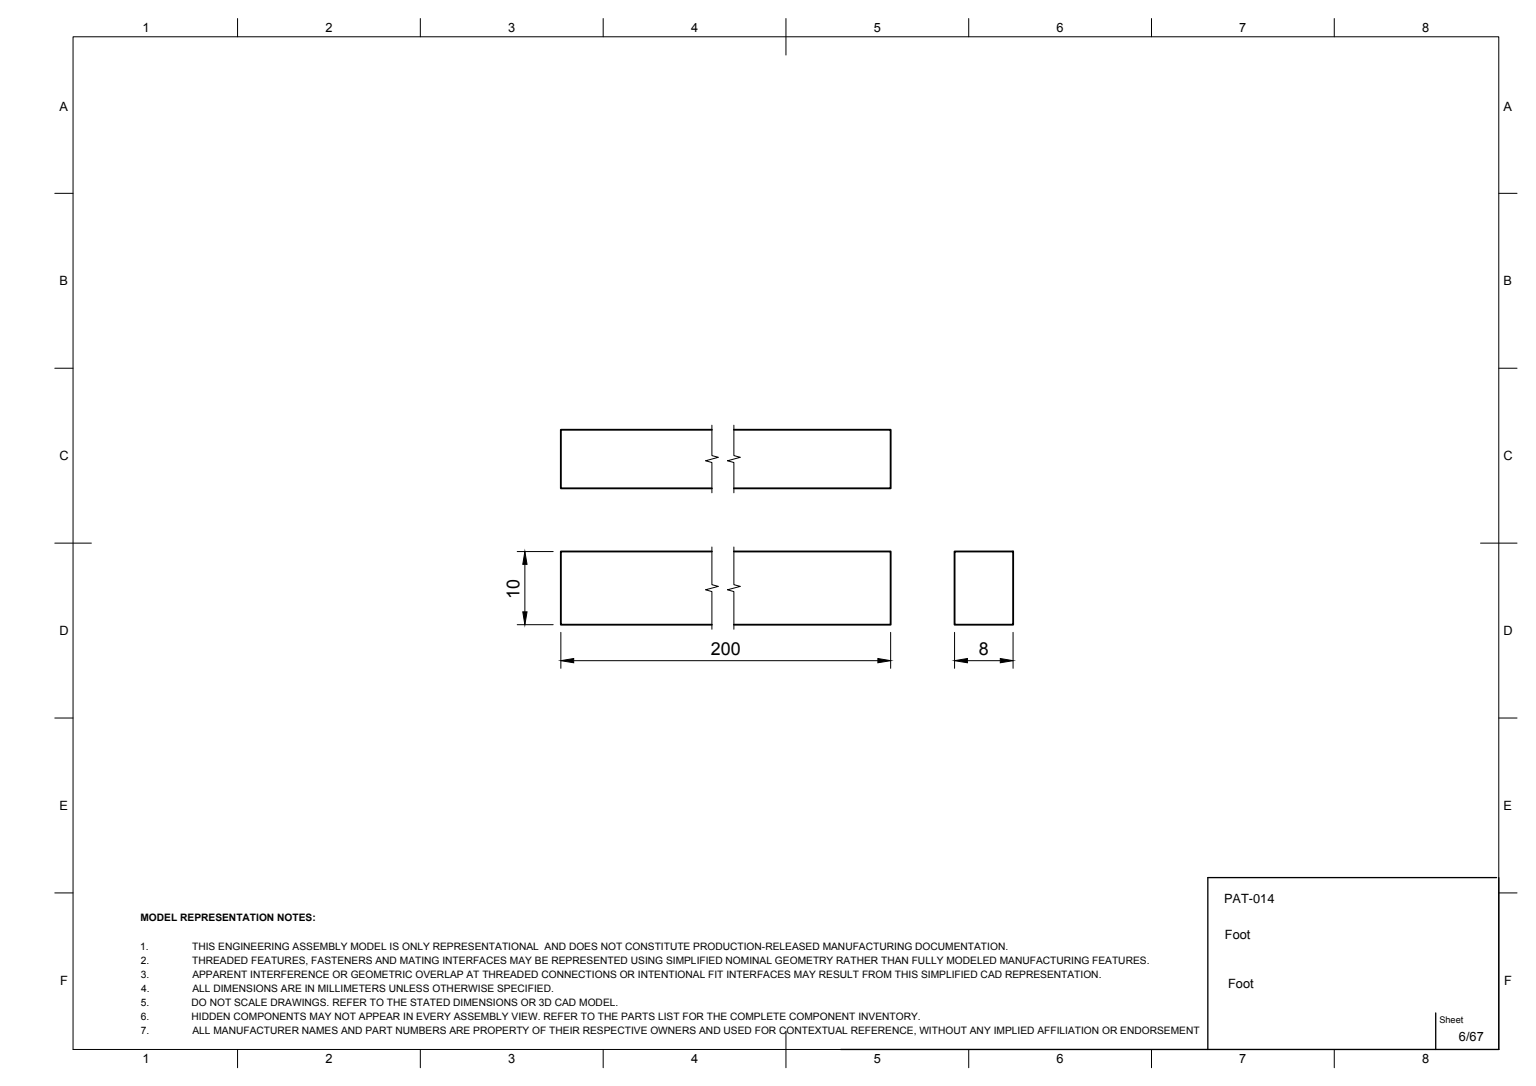
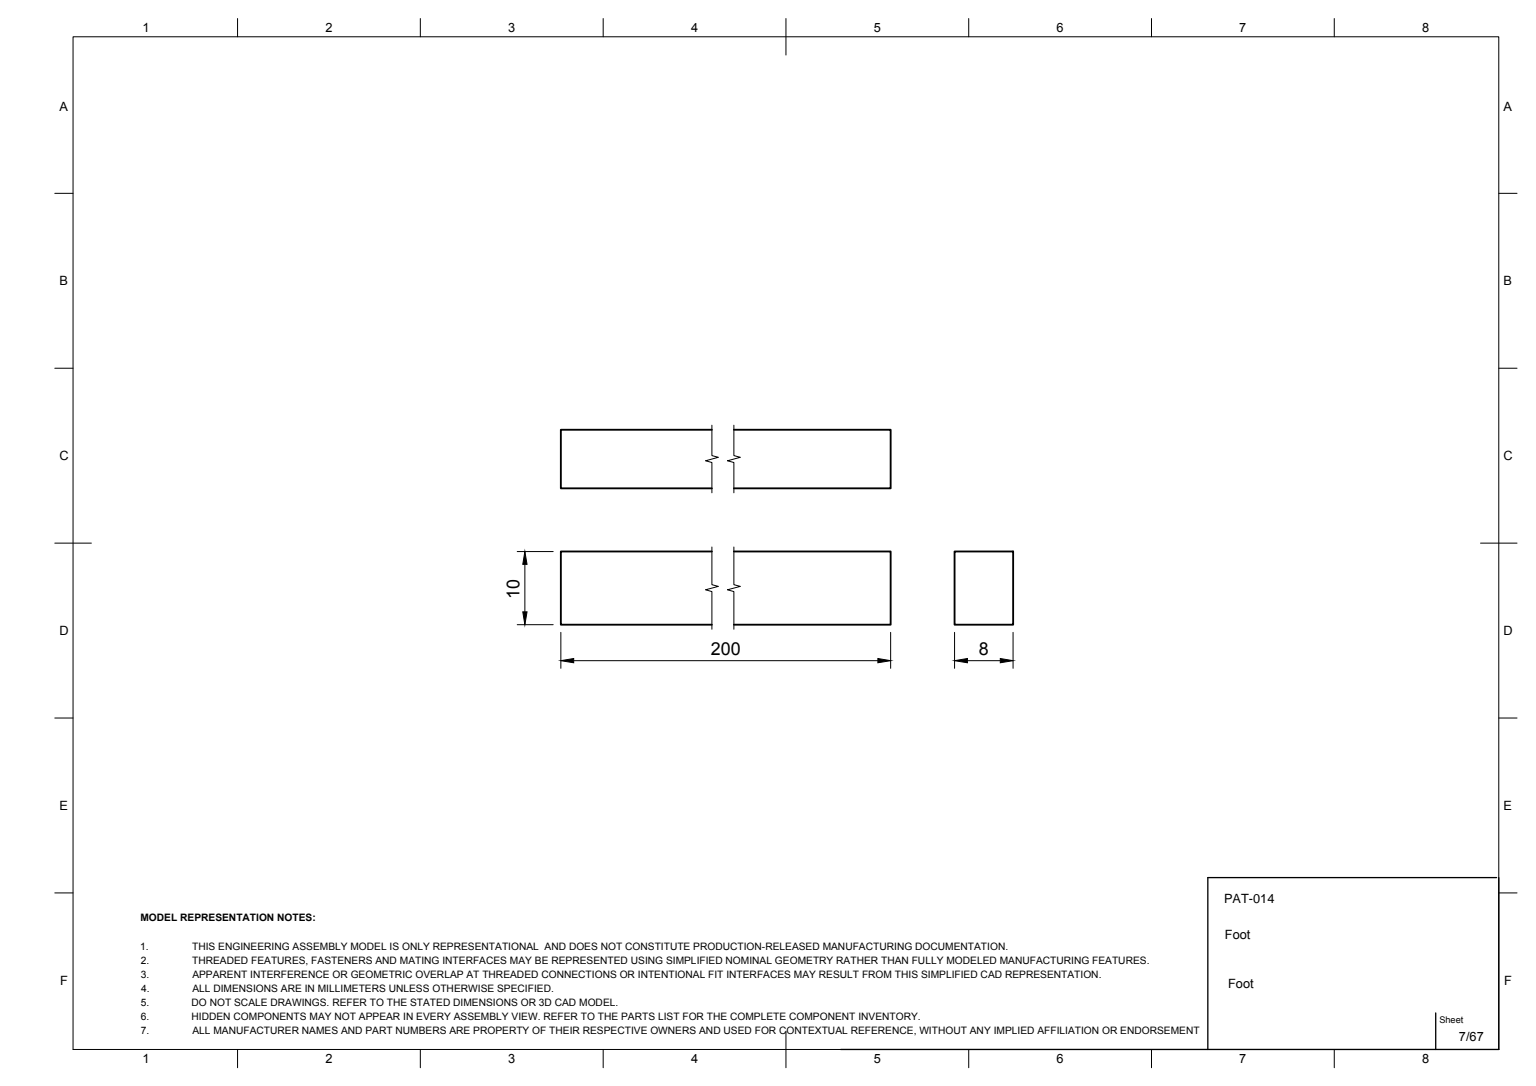
ISO-10303-21;
HEADER;
/* Generated by software containing ST-Developer
 * from STEP Tools, Inc. (www.steptools.com) 
 */

FILE_DESCRIPTION(
/* description */ ('Bin tilter linkage'),
/* implementation_level */ '2;1');

FILE_NAME(
/* name */ 'Foot.step',
/* time_stamp */ '2026-10-28T03:26:24-07:00',
/* author */ (''),
/* organization */ (''),
/* preprocessor_version */ 'ST-DEVELOPER v20.2',
/* originating_system */ 'Autodesk Translation Framework v15.17.0.0',
/* authorisation */ '');

FILE_SCHEMA (('AUTOMOTIVE_DESIGN { 1 0 10303 214 3 1 1 }'));
ENDSEC;

DATA;
#10=MECHANICAL_DESIGN_GEOMETRIC_PRESENTATION_REPRESENTATION('',(#863),#23728);
#651=SHAPE_REPRESENTATION_RELATIONSHIP('SRR','None',#24115,#757);
#757=ADVANCED_BREP_SHAPE_REPRESENTATION('',(#977),#23615);
#863=STYLED_ITEM('',(#24779),#977);
#977=MANIFOLD_SOLID_BREP('Body1',#12393);
#1498=PLANE('',#13722);
#1499=PLANE('',#13723);
#1500=PLANE('',#13724);
#1501=PLANE('',#13725);
#1502=PLANE('',#13726);
#1503=PLANE('',#13727);
#1908=FACE_OUTER_BOUND('',#2709,.T.);
#1909=FACE_OUTER_BOUND('',#2710,.T.);
#1910=FACE_OUTER_BOUND('',#2711,.T.);
#1911=FACE_OUTER_BOUND('',#2712,.T.);
#1912=FACE_OUTER_BOUND('',#2713,.T.);
#1913=FACE_OUTER_BOUND('',#2714,.T.);
#2709=EDGE_LOOP('',(#8469,#8470,#8471,#8472));
#2710=EDGE_LOOP('',(#8473,#8474,#8475,#8476));
#2711=EDGE_LOOP('',(#8477,#8478,#8479,#8480));
#2712=EDGE_LOOP('',(#8481,#8482,#8483,#8484));
#2713=EDGE_LOOP('',(#8485,#8486,#8487,#8488));
#2714=EDGE_LOOP('',(#8489,#8490,#8491,#8492));
#3873=LINE('',#19850,#4548);
#3874=LINE('',#19852,#4549);
#3875=LINE('',#19854,#4550);
#3876=LINE('',#19855,#4551);
#3877=LINE('',#19858,#4552);
#3878=LINE('',#19860,#4553);
#3879=LINE('',#19861,#4554);
#3880=LINE('',#19864,#4555);
#3881=LINE('',#19866,#4556);
#3882=LINE('',#19867,#4557);
#3883=LINE('',#19869,#4558);
#3884=LINE('',#19870,#4559);
#4548=VECTOR('',#15592,1.);
#4549=VECTOR('',#15593,1.);
#4550=VECTOR('',#15594,1.);
#4551=VECTOR('',#15595,1.);
#4552=VECTOR('',#15598,1.);
#4553=VECTOR('',#15599,1.);
#4554=VECTOR('',#15600,1.);
#4555=VECTOR('',#15603,1.);
#4556=VECTOR('',#15604,1.);
#4557=VECTOR('',#15605,1.);
#4558=VECTOR('',#15608,1.);
#4559=VECTOR('',#15609,1.);
#5989=VERTEX_POINT('',#19848);
#5990=VERTEX_POINT('',#19849);
#5991=VERTEX_POINT('',#19851);
#5992=VERTEX_POINT('',#19853);
#5993=VERTEX_POINT('',#19857);
#5994=VERTEX_POINT('',#19859);
#5995=VERTEX_POINT('',#19863);
#5996=VERTEX_POINT('',#19865);
#6974=EDGE_CURVE('',#5989,#5990,#3873,.T.);
#6975=EDGE_CURVE('',#5990,#5991,#3874,.T.);
#6976=EDGE_CURVE('',#5992,#5991,#3875,.T.);
#6977=EDGE_CURVE('',#5989,#5992,#3876,.T.);
#6978=EDGE_CURVE('',#5993,#5989,#3877,.T.);
#6979=EDGE_CURVE('',#5994,#5992,#3878,.T.);
#6980=EDGE_CURVE('',#5993,#5994,#3879,.T.);
#6981=EDGE_CURVE('',#5995,#5993,#3880,.T.);
#6982=EDGE_CURVE('',#5996,#5994,#3881,.T.);
#6983=EDGE_CURVE('',#5995,#5996,#3882,.T.);
#6984=EDGE_CURVE('',#5990,#5995,#3883,.T.);
#6985=EDGE_CURVE('',#5991,#5996,#3884,.T.);
#8469=ORIENTED_EDGE('',*,*,#6974,.T.);
#8470=ORIENTED_EDGE('',*,*,#6975,.T.);
#8471=ORIENTED_EDGE('',*,*,#6976,.F.);
#8472=ORIENTED_EDGE('',*,*,#6977,.F.);
#8473=ORIENTED_EDGE('',*,*,#6978,.T.);
#8474=ORIENTED_EDGE('',*,*,#6977,.T.);
#8475=ORIENTED_EDGE('',*,*,#6979,.F.);
#8476=ORIENTED_EDGE('',*,*,#6980,.F.);
#8477=ORIENTED_EDGE('',*,*,#6981,.T.);
#8478=ORIENTED_EDGE('',*,*,#6980,.T.);
#8479=ORIENTED_EDGE('',*,*,#6982,.F.);
#8480=ORIENTED_EDGE('',*,*,#6983,.F.);
#8481=ORIENTED_EDGE('',*,*,#6984,.T.);
#8482=ORIENTED_EDGE('',*,*,#6983,.T.);
#8483=ORIENTED_EDGE('',*,*,#6985,.F.);
#8484=ORIENTED_EDGE('',*,*,#6975,.F.);
#8485=ORIENTED_EDGE('',*,*,#6985,.T.);
#8486=ORIENTED_EDGE('',*,*,#6982,.T.);
#8487=ORIENTED_EDGE('',*,*,#6979,.T.);
#8488=ORIENTED_EDGE('',*,*,#6976,.T.);
#8489=ORIENTED_EDGE('',*,*,#6984,.F.);
#8490=ORIENTED_EDGE('',*,*,#6974,.F.);
#8491=ORIENTED_EDGE('',*,*,#6978,.F.);
#8492=ORIENTED_EDGE('',*,*,#6981,.F.);
#11633=ADVANCED_FACE('',(#1908),#1498,.T.);
#11634=ADVANCED_FACE('',(#1909),#1499,.T.);
#11635=ADVANCED_FACE('',(#1910),#1500,.T.);
#11636=ADVANCED_FACE('',(#1911),#1501,.T.);
#11637=ADVANCED_FACE('',(#1912),#1502,.T.);
#11638=ADVANCED_FACE('',(#1913),#1503,.F.);
#12393=CLOSED_SHELL('',(#11633,#11634,#11635,#11636,#11637,#11638));
#13721=AXIS2_PLACEMENT_3D('',#19846,#15588,#15589);
#13722=AXIS2_PLACEMENT_3D('',#19847,#15590,#15591);
#13723=AXIS2_PLACEMENT_3D('',#19856,#15596,#15597);
#13724=AXIS2_PLACEMENT_3D('',#19862,#15601,#15602);
#13725=AXIS2_PLACEMENT_3D('',#19868,#15606,#15607);
#13726=AXIS2_PLACEMENT_3D('',#19871,#15610,#15611);
#13727=AXIS2_PLACEMENT_3D('',#19872,#15612,#15613);
#15588=DIRECTION('axis',(0.,0.,1.));
#15589=DIRECTION('refdir',(1.,0.,0.));
#15590=DIRECTION('center_axis',(0.,1.,0.));
#15591=DIRECTION('ref_axis',(-1.,0.,0.));
#15592=DIRECTION('',(-1.,0.,0.));
#15593=DIRECTION('',(0.,0.,1.));
#15594=DIRECTION('',(-1.,0.,0.));
#15595=DIRECTION('',(0.,0.,1.));
#15596=DIRECTION('center_axis',(1.,0.,0.));
#15597=DIRECTION('ref_axis',(0.,1.,0.));
#15598=DIRECTION('',(0.,1.,0.));
#15599=DIRECTION('',(0.,1.,0.));
#15600=DIRECTION('',(0.,0.,1.));
#15601=DIRECTION('center_axis',(0.,-1.,0.));
#15602=DIRECTION('ref_axis',(1.,0.,0.));
#15603=DIRECTION('',(1.,0.,0.));
#15604=DIRECTION('',(1.,0.,0.));
#15605=DIRECTION('',(0.,0.,1.));
#15606=DIRECTION('center_axis',(-1.,0.,0.));
#15607=DIRECTION('ref_axis',(0.,-1.,0.));
#15608=DIRECTION('',(0.,-1.,0.));
#15609=DIRECTION('',(0.,-1.,0.));
#15610=DIRECTION('center_axis',(0.,0.,1.));
#15611=DIRECTION('ref_axis',(1.,0.,0.));
#15612=DIRECTION('center_axis',(0.,0.,1.));
#15613=DIRECTION('ref_axis',(1.,0.,0.));
#19846=CARTESIAN_POINT('',(0.,0.,0.));
#19847=CARTESIAN_POINT('Origin',(-13.,10.,-0.8));
#19848=CARTESIAN_POINT('',(-13.,10.,-0.8));
#19849=CARTESIAN_POINT('',(-14.,10.,-0.8));
#19850=CARTESIAN_POINT('',(-13.,10.,-0.8));
#19851=CARTESIAN_POINT('',(-14.,10.,0.));
#19852=CARTESIAN_POINT('',(-14.,10.,-0.8));
#19853=CARTESIAN_POINT('',(-13.,10.,0.));
#19854=CARTESIAN_POINT('',(-13.,10.,0.));
#19855=CARTESIAN_POINT('',(-13.,10.,-0.8));
#19856=CARTESIAN_POINT('Origin',(-13.,-10.,-0.8));
#19857=CARTESIAN_POINT('',(-13.,-10.,-0.8));
#19858=CARTESIAN_POINT('',(-13.,-10.,-0.8));
#19859=CARTESIAN_POINT('',(-13.,-10.,0.));
#19860=CARTESIAN_POINT('',(-13.,-10.,0.));
#19861=CARTESIAN_POINT('',(-13.,-10.,-0.8));
#19862=CARTESIAN_POINT('Origin',(-14.,-10.,-0.8));
#19863=CARTESIAN_POINT('',(-14.,-10.,-0.8));
#19864=CARTESIAN_POINT('',(-14.,-10.,-0.8));
#19865=CARTESIAN_POINT('',(-14.,-10.,0.));
#19866=CARTESIAN_POINT('',(-14.,-10.,0.));
#19867=CARTESIAN_POINT('',(-14.,-10.,-0.8));
#19868=CARTESIAN_POINT('Origin',(-14.,10.,-0.8));
#19869=CARTESIAN_POINT('',(-14.,10.,-0.8));
#19870=CARTESIAN_POINT('',(-14.,10.,0.));
#19871=CARTESIAN_POINT('Origin',(-13.5,0.,0.));
#19872=CARTESIAN_POINT('Origin',(-13.5,0.,-0.8));
#23498=UNCERTAINTY_MEASURE_WITH_UNIT(LENGTH_MEASURE(0.001),#23729,
'DISTANCE_ACCURACY_VALUE',
'Maximum model space distance between geometric entities at asserted c
onnectivities');
#23611=UNCERTAINTY_MEASURE_WITH_UNIT(LENGTH_MEASURE(0.001),#23729,
'DISTANCE_ACCURACY_VALUE',
'Maximum model space distance between geometric entities at asserted c
onnectivities');
#23615=(
GEOMETRIC_REPRESENTATION_CONTEXT(3)
GLOBAL_UNCERTAINTY_ASSIGNED_CONTEXT((#23498))
GLOBAL_UNIT_ASSIGNED_CONTEXT((#23729,#23731,#23732))
REPRESENTATION_CONTEXT('','3D')
);
#23728=(
GEOMETRIC_REPRESENTATION_CONTEXT(3)
GLOBAL_UNCERTAINTY_ASSIGNED_CONTEXT((#23611))
GLOBAL_UNIT_ASSIGNED_CONTEXT((#23729,#23731,#23732))
REPRESENTATION_CONTEXT('','3D')
);
#23729=(
LENGTH_UNIT()
NAMED_UNIT(*)
SI_UNIT(.CENTI.,.METRE.)
);
#23731=(
NAMED_UNIT(*)
PLANE_ANGLE_UNIT()
SI_UNIT($,.RADIAN.)
);
#23732=(
NAMED_UNIT(*)
SI_UNIT($,.STERADIAN.)
SOLID_ANGLE_UNIT()
);
#23736=SHAPE_DEFINITION_REPRESENTATION(#23852,#24115);
#23852=PRODUCT_DEFINITION_SHAPE('',$,#24232);
#24115=SHAPE_REPRESENTATION('',(#13721),#23615);
#24228=PRODUCT_DEFINITION_CONTEXT('part definition',#24578,'design');
#24232=PRODUCT_DEFINITION('Foot','Foot',#24348,#24228);
#24348=PRODUCT_DEFINITION_FORMATION('',$,#24583);
#24578=APPLICATION_CONTEXT(
'Core Data for Automotive Mechanical Design Process');
#24579=PRODUCT_CONTEXT('part definition',#24578,'mechanical');
#24583=PRODUCT('Foot','Foot','Foot',(#24579));
#24773=COLOUR_RGB('Off White',0.89,0.88,0.83);
#24774=FILL_AREA_STYLE_COLOUR('',#24773);
#24775=FILL_AREA_STYLE('',(#24774));
#24776=SURFACE_STYLE_FILL_AREA(#24775);
#24777=SURFACE_SIDE_STYLE('',(#24776));
#24778=SURFACE_STYLE_USAGE(.BOTH.,#24777);
#24779=PRESENTATION_STYLE_ASSIGNMENT((#24778));
ENDSEC;
END-ISO-10303-21;
